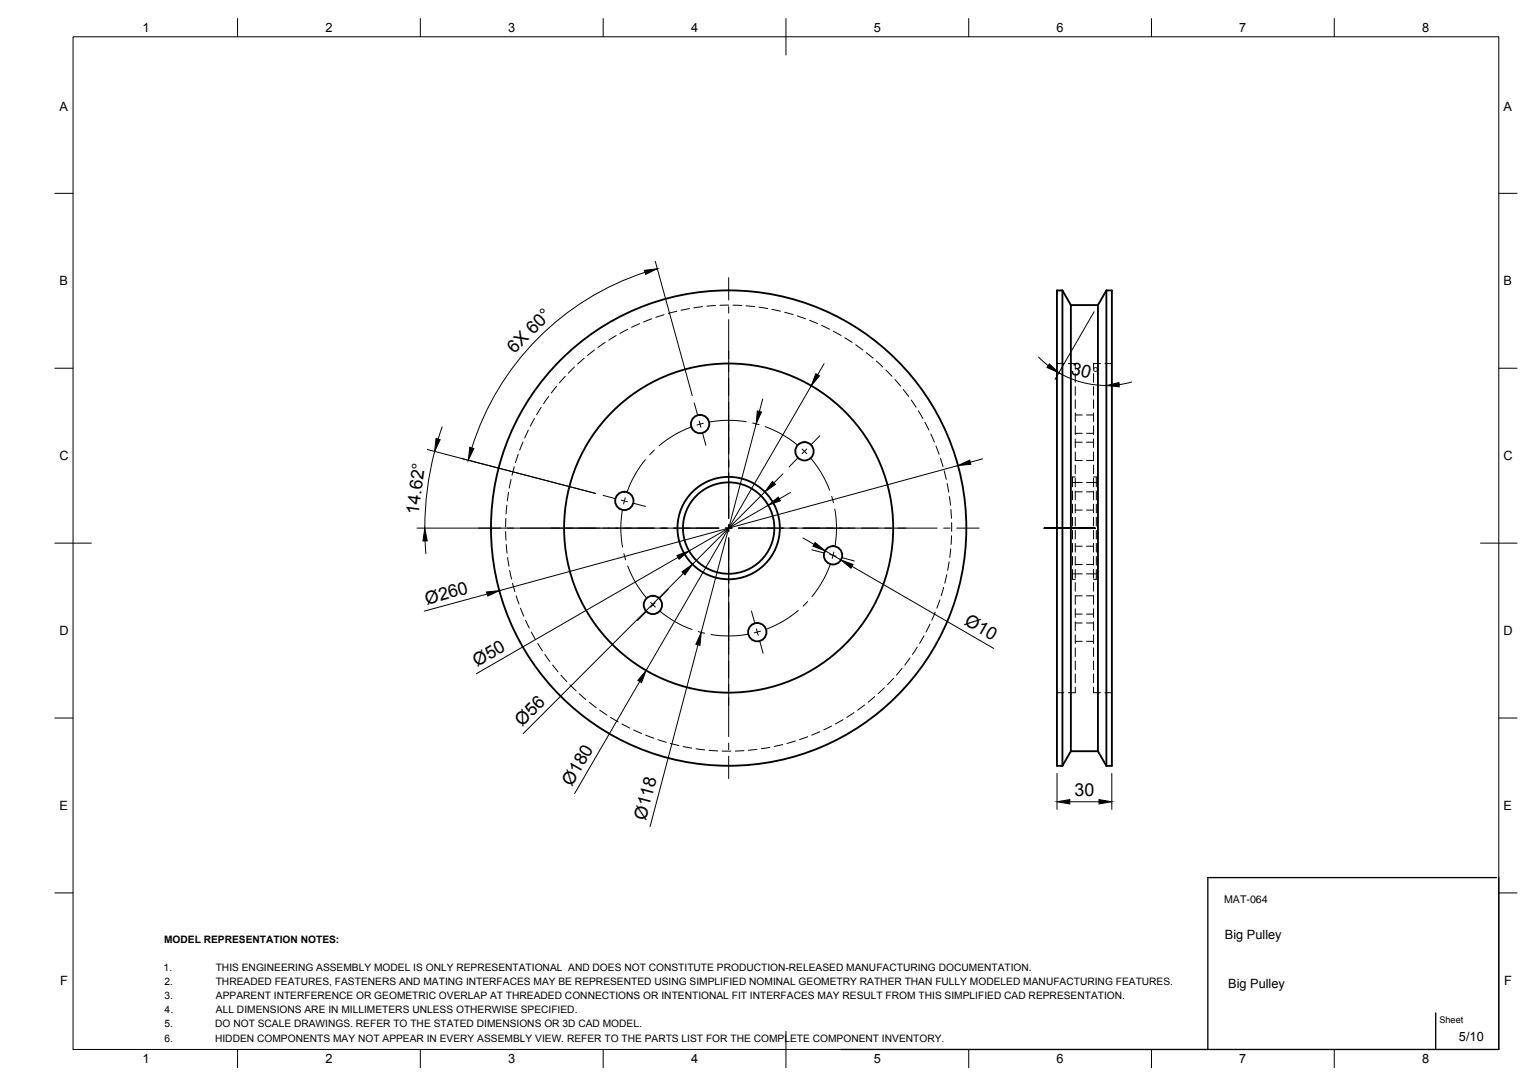
ISO-10303-21;
HEADER;
/* Generated by software containing ST-Developer
 * from STEP Tools, Inc. (www.steptools.com) 
 */

FILE_DESCRIPTION(
/* description */ (''),
/* implementation_level */ '2;1');

FILE_NAME(
/* name */ 
'Big Pulley.step',
/* time_stamp */ '2026-10-24T12:42:14-07:00',
/* author */ (''),
/* organization */ (''),
/* preprocessor_version */ 'ST-DEVELOPER v20.2',
/* originating_system */ 'Autodesk Translation Framework v15.15.0.0',
/* authorisation */ '');

FILE_SCHEMA (('AUTOMOTIVE_DESIGN { 1 0 10303 214 3 1 1 }'));
ENDSEC;

DATA;
#10=MECHANICAL_DESIGN_GEOMETRIC_PRESENTATION_REPRESENTATION('',(#70),#6789);
#16=CONICAL_SURFACE('',#4399,122.,1.04719755119659);
#17=CONICAL_SURFACE('',#4402,130.,1.04719755119659);
#58=SHAPE_REPRESENTATION_RELATIONSHIP('SRR','None',#6825,#64);
#64=ADVANCED_BREP_SHAPE_REPRESENTATION('',(#76),#6787);
#70=STYLED_ITEM('',(#6864),#76);
#76=MANIFOLD_SOLID_BREP('Big Pulley',#3965);
#167=CYLINDRICAL_SURFACE('',#4353,130.);
#168=CYLINDRICAL_SURFACE('',#4356,130.);
#169=CYLINDRICAL_SURFACE('',#4360,5.);
#170=CYLINDRICAL_SURFACE('',#4363,5.);
#171=CYLINDRICAL_SURFACE('',#4366,5.);
#172=CYLINDRICAL_SURFACE('',#4369,5.);
#173=CYLINDRICAL_SURFACE('',#4372,5.);
#174=CYLINDRICAL_SURFACE('',#4375,90.);
#175=CYLINDRICAL_SURFACE('',#4378,90.);
#176=CYLINDRICAL_SURFACE('',#4389,28.);
#177=CYLINDRICAL_SURFACE('',#4391,25.);
#178=CYLINDRICAL_SURFACE('',#4394,28.);
#179=CYLINDRICAL_SURFACE('',#4398,5.);
#180=CYLINDRICAL_SURFACE('',#4404,122.);
#224=FACE_BOUND('',#839,.T.);
#225=FACE_BOUND('',#841,.T.);
#226=FACE_BOUND('',#843,.T.);
#227=FACE_BOUND('',#844,.T.);
#228=FACE_BOUND('',#845,.T.);
#229=FACE_BOUND('',#846,.T.);
#230=FACE_BOUND('',#847,.T.);
#231=FACE_BOUND('',#848,.T.);
#232=FACE_BOUND('',#849,.T.);
#233=FACE_BOUND('',#851,.T.);
#234=FACE_BOUND('',#852,.T.);
#235=FACE_BOUND('',#853,.T.);
#236=FACE_BOUND('',#854,.T.);
#237=FACE_BOUND('',#855,.T.);
#238=FACE_BOUND('',#856,.T.);
#239=FACE_BOUND('',#857,.T.);
#240=FACE_BOUND('',#862,.T.);
#241=FACE_BOUND('',#864,.T.);
#356=CIRCLE('',#4354,130.);
#357=CIRCLE('',#4355,130.);
#358=CIRCLE('',#4357,130.);
#359=CIRCLE('',#4358,130.);
#360=CIRCLE('',#4359,130.);
#361=CIRCLE('',#4361,5.);
#362=CIRCLE('',#4362,5.);
#363=CIRCLE('',#4364,5.);
#364=CIRCLE('',#4365,5.);
#365=CIRCLE('',#4367,5.);
#366=CIRCLE('',#4368,5.);
#367=CIRCLE('',#4370,5.);
#368=CIRCLE('',#4371,5.);
#369=CIRCLE('',#4373,5.);
#370=CIRCLE('',#4374,5.);
#371=CIRCLE('',#4376,90.);
#372=CIRCLE('',#4377,90.);
#373=CIRCLE('',#4379,90.);
#374=CIRCLE('',#4380,90.);
#375=CIRCLE('',#4384,5.);
#376=CIRCLE('',#4385,28.);
#377=CIRCLE('',#4387,5.);
#378=CIRCLE('',#4388,28.);
#379=CIRCLE('',#4390,28.);
#380=CIRCLE('',#4392,25.);
#381=CIRCLE('',#4393,25.);
#382=CIRCLE('',#4395,28.);
#383=CIRCLE('',#4400,122.);
#384=CIRCLE('',#4401,122.);
#385=CIRCLE('',#4403,122.);
#573=FACE_OUTER_BOUND('',#829,.T.);
#574=FACE_OUTER_BOUND('',#830,.T.);
#575=FACE_OUTER_BOUND('',#831,.T.);
#576=FACE_OUTER_BOUND('',#832,.T.);
#577=FACE_OUTER_BOUND('',#833,.T.);
#578=FACE_OUTER_BOUND('',#834,.T.);
#579=FACE_OUTER_BOUND('',#835,.T.);
#580=FACE_OUTER_BOUND('',#836,.T.);
#581=FACE_OUTER_BOUND('',#837,.T.);
#582=FACE_OUTER_BOUND('',#838,.T.);
#583=FACE_OUTER_BOUND('',#840,.T.);
#584=FACE_OUTER_BOUND('',#842,.T.);
#585=FACE_OUTER_BOUND('',#850,.T.);
#586=FACE_OUTER_BOUND('',#858,.T.);
#587=FACE_OUTER_BOUND('',#859,.T.);
#588=FACE_OUTER_BOUND('',#860,.T.);
#589=FACE_OUTER_BOUND('',#861,.T.);
#590=FACE_OUTER_BOUND('',#863,.T.);
#591=FACE_OUTER_BOUND('',#865,.T.);
#592=FACE_OUTER_BOUND('',#866,.T.);
#593=FACE_OUTER_BOUND('',#867,.T.);
#594=FACE_OUTER_BOUND('',#868,.T.);
#829=EDGE_LOOP('',(#3469,#3470,#3471,#3472));
#830=EDGE_LOOP('',(#3473,#3474,#3475,#3476,#3477));
#831=EDGE_LOOP('',(#3478,#3479,#3480,#3481));
#832=EDGE_LOOP('',(#3482,#3483,#3484,#3485));
#833=EDGE_LOOP('',(#3486,#3487,#3488,#3489));
#834=EDGE_LOOP('',(#3490,#3491,#3492,#3493));
#835=EDGE_LOOP('',(#3494,#3495,#3496,#3497));
#836=EDGE_LOOP('',(#3498,#3499,#3500,#3501));
#837=EDGE_LOOP('',(#3502,#3503,#3504,#3505));
#838=EDGE_LOOP('',(#3506));
#839=EDGE_LOOP('',(#3507));
#840=EDGE_LOOP('',(#3508));
#841=EDGE_LOOP('',(#3509));
#842=EDGE_LOOP('',(#3510));
#843=EDGE_LOOP('',(#3511));
#844=EDGE_LOOP('',(#3512));
#845=EDGE_LOOP('',(#3513));
#846=EDGE_LOOP('',(#3514));
#847=EDGE_LOOP('',(#3515));
#848=EDGE_LOOP('',(#3516));
#849=EDGE_LOOP('',(#3517));
#850=EDGE_LOOP('',(#3518));
#851=EDGE_LOOP('',(#3519));
#852=EDGE_LOOP('',(#3520));
#853=EDGE_LOOP('',(#3521));
#854=EDGE_LOOP('',(#3522));
#855=EDGE_LOOP('',(#3523));
#856=EDGE_LOOP('',(#3524));
#857=EDGE_LOOP('',(#3525));
#858=EDGE_LOOP('',(#3526,#3527,#3528,#3529));
#859=EDGE_LOOP('',(#3530,#3531,#3532,#3533));
#860=EDGE_LOOP('',(#3534,#3535,#3536,#3537));
#861=EDGE_LOOP('',(#3538));
#862=EDGE_LOOP('',(#3539));
#863=EDGE_LOOP('',(#3540));
#864=EDGE_LOOP('',(#3541));
#865=EDGE_LOOP('',(#3542,#3543,#3544,#3545));
#866=EDGE_LOOP('',(#3546,#3547,#3548,#3549,#3550));
#867=EDGE_LOOP('',(#3551,#3552,#3553,#3554,#3555));
#868=EDGE_LOOP('',(#3556,#3557,#3558,#3559,#3560));
#1223=LINE('',#6567,#1601);
#1224=LINE('',#6575,#1602);
#1225=LINE('',#6581,#1603);
#1226=LINE('',#6587,#1604);
#1227=LINE('',#6593,#1605);
#1228=LINE('',#6599,#1606);
#1229=LINE('',#6605,#1607);
#1230=LINE('',#6611,#1608);
#1231=LINE('',#6617,#1609);
#1232=LINE('',#6634,#1610);
#1233=LINE('',#6639,#1611);
#1234=LINE('',#6643,#1612);
#1235=LINE('',#6648,#1613);
#1236=LINE('',#6651,#1614);
#1237=LINE('',#6657,#1615);
#1238=LINE('',#6660,#1616);
#1601=VECTOR('',#5412,130.);
#1602=VECTOR('',#5421,130.);
#1603=VECTOR('',#5428,5.);
#1604=VECTOR('',#5435,5.);
#1605=VECTOR('',#5442,5.);
#1606=VECTOR('',#5449,5.);
#1607=VECTOR('',#5456,5.);
#1608=VECTOR('',#5463,90.);
#1609=VECTOR('',#5470,90.);
#1610=VECTOR('',#5493,28.);
#1611=VECTOR('',#5498,25.);
#1612=VECTOR('',#5503,28.);
#1613=VECTOR('',#5512,5.);
#1614=VECTOR('',#5515,122.);
#1615=VECTOR('',#5522,130.);
#1616=VECTOR('',#5527,122.);
#1941=VERTEX_POINT('',#6564);
#1942=VERTEX_POINT('',#6566);
#1943=VERTEX_POINT('',#6570);
#1944=VERTEX_POINT('',#6571);
#1945=VERTEX_POINT('',#6574);
#1946=VERTEX_POINT('',#6578);
#1947=VERTEX_POINT('',#6580);
#1948=VERTEX_POINT('',#6584);
#1949=VERTEX_POINT('',#6586);
#1950=VERTEX_POINT('',#6590);
#1951=VERTEX_POINT('',#6592);
#1952=VERTEX_POINT('',#6596);
#1953=VERTEX_POINT('',#6598);
#1954=VERTEX_POINT('',#6602);
#1955=VERTEX_POINT('',#6604);
#1956=VERTEX_POINT('',#6608);
#1957=VERTEX_POINT('',#6610);
#1958=VERTEX_POINT('',#6614);
#1959=VERTEX_POINT('',#6616);
#1960=VERTEX_POINT('',#6622);
#1961=VERTEX_POINT('',#6624);
#1962=VERTEX_POINT('',#6627);
#1963=VERTEX_POINT('',#6629);
#1964=VERTEX_POINT('',#6632);
#1965=VERTEX_POINT('',#6636);
#1966=VERTEX_POINT('',#6638);
#1967=VERTEX_POINT('',#6642);
#1968=VERTEX_POINT('',#6650);
#1969=VERTEX_POINT('',#6652);
#1970=VERTEX_POINT('',#6656);
#2455=EDGE_CURVE('',#1941,#1941,#356,.T.);
#2456=EDGE_CURVE('',#1941,#1942,#1223,.T.);
#2457=EDGE_CURVE('',#1942,#1942,#357,.T.);
#2458=EDGE_CURVE('',#1943,#1944,#358,.T.);
#2459=EDGE_CURVE('',#1944,#1943,#359,.T.);
#2460=EDGE_CURVE('',#1943,#1945,#1224,.T.);
#2461=EDGE_CURVE('',#1945,#1945,#360,.T.);
#2462=EDGE_CURVE('',#1946,#1946,#361,.T.);
#2463=EDGE_CURVE('',#1946,#1947,#1225,.T.);
#2464=EDGE_CURVE('',#1947,#1947,#362,.T.);
#2465=EDGE_CURVE('',#1948,#1948,#363,.T.);
#2466=EDGE_CURVE('',#1948,#1949,#1226,.T.);
#2467=EDGE_CURVE('',#1949,#1949,#364,.T.);
#2468=EDGE_CURVE('',#1950,#1950,#365,.T.);
#2469=EDGE_CURVE('',#1950,#1951,#1227,.T.);
#2470=EDGE_CURVE('',#1951,#1951,#366,.T.);
#2471=EDGE_CURVE('',#1952,#1952,#367,.T.);
#2472=EDGE_CURVE('',#1952,#1953,#1228,.T.);
#2473=EDGE_CURVE('',#1953,#1953,#368,.T.);
#2474=EDGE_CURVE('',#1954,#1954,#369,.T.);
#2475=EDGE_CURVE('',#1954,#1955,#1229,.T.);
#2476=EDGE_CURVE('',#1955,#1955,#370,.T.);
#2477=EDGE_CURVE('',#1956,#1956,#371,.T.);
#2478=EDGE_CURVE('',#1956,#1957,#1230,.T.);
#2479=EDGE_CURVE('',#1957,#1957,#372,.T.);
#2480=EDGE_CURVE('',#1958,#1958,#373,.T.);
#2481=EDGE_CURVE('',#1958,#1959,#1231,.T.);
#2482=EDGE_CURVE('',#1959,#1959,#374,.T.);
#2483=EDGE_CURVE('',#1960,#1960,#375,.T.);
#2484=EDGE_CURVE('',#1961,#1961,#376,.T.);
#2485=EDGE_CURVE('',#1962,#1962,#377,.T.);
#2486=EDGE_CURVE('',#1963,#1963,#378,.F.);
#2487=EDGE_CURVE('',#1964,#1964,#379,.T.);
#2488=EDGE_CURVE('',#1964,#1963,#1232,.T.);
#2489=EDGE_CURVE('',#1965,#1965,#380,.T.);
#2490=EDGE_CURVE('',#1965,#1966,#1233,.T.);
#2491=EDGE_CURVE('',#1966,#1966,#381,.T.);
#2492=EDGE_CURVE('',#1961,#1967,#1234,.T.);
#2493=EDGE_CURVE('',#1967,#1967,#382,.T.);
#2494=EDGE_CURVE('',#1962,#1960,#1235,.T.);
#2495=EDGE_CURVE('',#1942,#1968,#1236,.T.);
#2496=EDGE_CURVE('',#1969,#1968,#383,.T.);
#2497=EDGE_CURVE('',#1968,#1969,#384,.T.);
#2498=EDGE_CURVE('',#1944,#1970,#1237,.T.);
#2499=EDGE_CURVE('',#1970,#1970,#385,.T.);
#2500=EDGE_CURVE('',#1970,#1969,#1238,.T.);
#3469=ORIENTED_EDGE('',*,*,#2455,.T.);
#3470=ORIENTED_EDGE('',*,*,#2456,.T.);
#3471=ORIENTED_EDGE('',*,*,#2457,.F.);
#3472=ORIENTED_EDGE('',*,*,#2456,.F.);
#3473=ORIENTED_EDGE('',*,*,#2458,.T.);
#3474=ORIENTED_EDGE('',*,*,#2459,.T.);
#3475=ORIENTED_EDGE('',*,*,#2460,.T.);
#3476=ORIENTED_EDGE('',*,*,#2461,.F.);
#3477=ORIENTED_EDGE('',*,*,#2460,.F.);
#3478=ORIENTED_EDGE('',*,*,#2462,.F.);
#3479=ORIENTED_EDGE('',*,*,#2463,.T.);
#3480=ORIENTED_EDGE('',*,*,#2464,.T.);
#3481=ORIENTED_EDGE('',*,*,#2463,.F.);
#3482=ORIENTED_EDGE('',*,*,#2465,.F.);
#3483=ORIENTED_EDGE('',*,*,#2466,.T.);
#3484=ORIENTED_EDGE('',*,*,#2467,.T.);
#3485=ORIENTED_EDGE('',*,*,#2466,.F.);
#3486=ORIENTED_EDGE('',*,*,#2468,.F.);
#3487=ORIENTED_EDGE('',*,*,#2469,.T.);
#3488=ORIENTED_EDGE('',*,*,#2470,.T.);
#3489=ORIENTED_EDGE('',*,*,#2469,.F.);
#3490=ORIENTED_EDGE('',*,*,#2471,.F.);
#3491=ORIENTED_EDGE('',*,*,#2472,.T.);
#3492=ORIENTED_EDGE('',*,*,#2473,.T.);
#3493=ORIENTED_EDGE('',*,*,#2472,.F.);
#3494=ORIENTED_EDGE('',*,*,#2474,.F.);
#3495=ORIENTED_EDGE('',*,*,#2475,.T.);
#3496=ORIENTED_EDGE('',*,*,#2476,.T.);
#3497=ORIENTED_EDGE('',*,*,#2475,.F.);
#3498=ORIENTED_EDGE('',*,*,#2477,.T.);
#3499=ORIENTED_EDGE('',*,*,#2478,.T.);
#3500=ORIENTED_EDGE('',*,*,#2479,.F.);
#3501=ORIENTED_EDGE('',*,*,#2478,.F.);
#3502=ORIENTED_EDGE('',*,*,#2480,.T.);
#3503=ORIENTED_EDGE('',*,*,#2481,.T.);
#3504=ORIENTED_EDGE('',*,*,#2482,.F.);
#3505=ORIENTED_EDGE('',*,*,#2481,.F.);
#3506=ORIENTED_EDGE('',*,*,#2461,.T.);
#3507=ORIENTED_EDGE('',*,*,#2480,.F.);
#3508=ORIENTED_EDGE('',*,*,#2455,.F.);
#3509=ORIENTED_EDGE('',*,*,#2479,.T.);
#3510=ORIENTED_EDGE('',*,*,#2482,.T.);
#3511=ORIENTED_EDGE('',*,*,#2464,.F.);
#3512=ORIENTED_EDGE('',*,*,#2467,.F.);
#3513=ORIENTED_EDGE('',*,*,#2470,.F.);
#3514=ORIENTED_EDGE('',*,*,#2473,.F.);
#3515=ORIENTED_EDGE('',*,*,#2476,.F.);
#3516=ORIENTED_EDGE('',*,*,#2483,.F.);
#3517=ORIENTED_EDGE('',*,*,#2484,.F.);
#3518=ORIENTED_EDGE('',*,*,#2477,.F.);
#3519=ORIENTED_EDGE('',*,*,#2462,.T.);
#3520=ORIENTED_EDGE('',*,*,#2465,.T.);
#3521=ORIENTED_EDGE('',*,*,#2468,.T.);
#3522=ORIENTED_EDGE('',*,*,#2471,.T.);
#3523=ORIENTED_EDGE('',*,*,#2474,.T.);
#3524=ORIENTED_EDGE('',*,*,#2485,.T.);
#3525=ORIENTED_EDGE('',*,*,#2486,.F.);
#3526=ORIENTED_EDGE('',*,*,#2487,.T.);
#3527=ORIENTED_EDGE('',*,*,#2488,.T.);
#3528=ORIENTED_EDGE('',*,*,#2486,.T.);
#3529=ORIENTED_EDGE('',*,*,#2488,.F.);
#3530=ORIENTED_EDGE('',*,*,#2489,.T.);
#3531=ORIENTED_EDGE('',*,*,#2490,.T.);
#3532=ORIENTED_EDGE('',*,*,#2491,.F.);
#3533=ORIENTED_EDGE('',*,*,#2490,.F.);
#3534=ORIENTED_EDGE('',*,*,#2484,.T.);
#3535=ORIENTED_EDGE('',*,*,#2492,.T.);
#3536=ORIENTED_EDGE('',*,*,#2493,.F.);
#3537=ORIENTED_EDGE('',*,*,#2492,.F.);
#3538=ORIENTED_EDGE('',*,*,#2493,.T.);
#3539=ORIENTED_EDGE('',*,*,#2489,.F.);
#3540=ORIENTED_EDGE('',*,*,#2487,.F.);
#3541=ORIENTED_EDGE('',*,*,#2491,.T.);
#3542=ORIENTED_EDGE('',*,*,#2485,.F.);
#3543=ORIENTED_EDGE('',*,*,#2494,.T.);
#3544=ORIENTED_EDGE('',*,*,#2483,.T.);
#3545=ORIENTED_EDGE('',*,*,#2494,.F.);
#3546=ORIENTED_EDGE('',*,*,#2457,.T.);
#3547=ORIENTED_EDGE('',*,*,#2495,.T.);
#3548=ORIENTED_EDGE('',*,*,#2496,.F.);
#3549=ORIENTED_EDGE('',*,*,#2497,.F.);
#3550=ORIENTED_EDGE('',*,*,#2495,.F.);
#3551=ORIENTED_EDGE('',*,*,#2458,.F.);
#3552=ORIENTED_EDGE('',*,*,#2459,.F.);
#3553=ORIENTED_EDGE('',*,*,#2498,.T.);
#3554=ORIENTED_EDGE('',*,*,#2499,.T.);
#3555=ORIENTED_EDGE('',*,*,#2498,.F.);
#3556=ORIENTED_EDGE('',*,*,#2499,.F.);
#3557=ORIENTED_EDGE('',*,*,#2500,.T.);
#3558=ORIENTED_EDGE('',*,*,#2496,.T.);
#3559=ORIENTED_EDGE('',*,*,#2497,.T.);
#3560=ORIENTED_EDGE('',*,*,#2500,.F.);
#3730=PLANE('',#4381);
#3731=PLANE('',#4382);
#3732=PLANE('',#4383);
#3733=PLANE('',#4386);
#3734=PLANE('',#4396);
#3735=PLANE('',#4397);
#3923=ADVANCED_FACE('',(#573),#167,.T.);
#3924=ADVANCED_FACE('',(#574),#168,.T.);
#3925=ADVANCED_FACE('',(#575),#169,.F.);
#3926=ADVANCED_FACE('',(#576),#170,.F.);
#3927=ADVANCED_FACE('',(#577),#171,.F.);
#3928=ADVANCED_FACE('',(#578),#172,.F.);
#3929=ADVANCED_FACE('',(#579),#173,.F.);
#3930=ADVANCED_FACE('',(#580),#174,.F.);
#3931=ADVANCED_FACE('',(#581),#175,.F.);
#3932=ADVANCED_FACE('',(#582,#224),#3730,.T.);
#3933=ADVANCED_FACE('',(#583,#225),#3731,.F.);
#3934=ADVANCED_FACE('',(#584,#226,#227,#228,#229,#230,#231,#232),#3732,
 .T.);
#3935=ADVANCED_FACE('',(#585,#233,#234,#235,#236,#237,#238,#239),#3733,
 .F.);
#3936=ADVANCED_FACE('',(#586),#176,.T.);
#3937=ADVANCED_FACE('',(#587),#177,.F.);
#3938=ADVANCED_FACE('',(#588),#178,.T.);
#3939=ADVANCED_FACE('',(#589,#240),#3734,.T.);
#3940=ADVANCED_FACE('',(#590,#241),#3735,.F.);
#3941=ADVANCED_FACE('',(#591),#179,.F.);
#3942=ADVANCED_FACE('',(#592),#16,.T.);
#3943=ADVANCED_FACE('',(#593),#17,.T.);
#3944=ADVANCED_FACE('',(#594),#180,.T.);
#3965=CLOSED_SHELL('',(#3923,#3924,#3925,#3926,#3927,#3928,#3929,#3930,
#3931,#3932,#3933,#3934,#3935,#3936,#3937,#3938,#3939,#3940,#3941,#3942,
#3943,#3944));
#4352=AXIS2_PLACEMENT_3D('',#6562,#5406,#5407);
#4353=AXIS2_PLACEMENT_3D('',#6563,#5408,#5409);
#4354=AXIS2_PLACEMENT_3D('',#6565,#5410,#5411);
#4355=AXIS2_PLACEMENT_3D('',#6568,#5413,#5414);
#4356=AXIS2_PLACEMENT_3D('',#6569,#5415,#5416);
#4357=AXIS2_PLACEMENT_3D('',#6572,#5417,#5418);
#4358=AXIS2_PLACEMENT_3D('',#6573,#5419,#5420);
#4359=AXIS2_PLACEMENT_3D('',#6576,#5422,#5423);
#4360=AXIS2_PLACEMENT_3D('',#6577,#5424,#5425);
#4361=AXIS2_PLACEMENT_3D('',#6579,#5426,#5427);
#4362=AXIS2_PLACEMENT_3D('',#6582,#5429,#5430);
#4363=AXIS2_PLACEMENT_3D('',#6583,#5431,#5432);
#4364=AXIS2_PLACEMENT_3D('',#6585,#5433,#5434);
#4365=AXIS2_PLACEMENT_3D('',#6588,#5436,#5437);
#4366=AXIS2_PLACEMENT_3D('',#6589,#5438,#5439);
#4367=AXIS2_PLACEMENT_3D('',#6591,#5440,#5441);
#4368=AXIS2_PLACEMENT_3D('',#6594,#5443,#5444);
#4369=AXIS2_PLACEMENT_3D('',#6595,#5445,#5446);
#4370=AXIS2_PLACEMENT_3D('',#6597,#5447,#5448);
#4371=AXIS2_PLACEMENT_3D('',#6600,#5450,#5451);
#4372=AXIS2_PLACEMENT_3D('',#6601,#5452,#5453);
#4373=AXIS2_PLACEMENT_3D('',#6603,#5454,#5455);
#4374=AXIS2_PLACEMENT_3D('',#6606,#5457,#5458);
#4375=AXIS2_PLACEMENT_3D('',#6607,#5459,#5460);
#4376=AXIS2_PLACEMENT_3D('',#6609,#5461,#5462);
#4377=AXIS2_PLACEMENT_3D('',#6612,#5464,#5465);
#4378=AXIS2_PLACEMENT_3D('',#6613,#5466,#5467);
#4379=AXIS2_PLACEMENT_3D('',#6615,#5468,#5469);
#4380=AXIS2_PLACEMENT_3D('',#6618,#5471,#5472);
#4381=AXIS2_PLACEMENT_3D('',#6619,#5473,#5474);
#4382=AXIS2_PLACEMENT_3D('',#6620,#5475,#5476);
#4383=AXIS2_PLACEMENT_3D('',#6621,#5477,#5478);
#4384=AXIS2_PLACEMENT_3D('',#6623,#5479,#5480);
#4385=AXIS2_PLACEMENT_3D('',#6625,#5481,#5482);
#4386=AXIS2_PLACEMENT_3D('',#6626,#5483,#5484);
#4387=AXIS2_PLACEMENT_3D('',#6628,#5485,#5486);
#4388=AXIS2_PLACEMENT_3D('',#6630,#5487,#5488);
#4389=AXIS2_PLACEMENT_3D('',#6631,#5489,#5490);
#4390=AXIS2_PLACEMENT_3D('',#6633,#5491,#5492);
#4391=AXIS2_PLACEMENT_3D('',#6635,#5494,#5495);
#4392=AXIS2_PLACEMENT_3D('',#6637,#5496,#5497);
#4393=AXIS2_PLACEMENT_3D('',#6640,#5499,#5500);
#4394=AXIS2_PLACEMENT_3D('',#6641,#5501,#5502);
#4395=AXIS2_PLACEMENT_3D('',#6644,#5504,#5505);
#4396=AXIS2_PLACEMENT_3D('',#6645,#5506,#5507);
#4397=AXIS2_PLACEMENT_3D('',#6646,#5508,#5509);
#4398=AXIS2_PLACEMENT_3D('',#6647,#5510,#5511);
#4399=AXIS2_PLACEMENT_3D('',#6649,#5513,#5514);
#4400=AXIS2_PLACEMENT_3D('',#6653,#5516,#5517);
#4401=AXIS2_PLACEMENT_3D('',#6654,#5518,#5519);
#4402=AXIS2_PLACEMENT_3D('',#6655,#5520,#5521);
#4403=AXIS2_PLACEMENT_3D('',#6658,#5523,#5524);
#4404=AXIS2_PLACEMENT_3D('',#6659,#5525,#5526);
#5406=DIRECTION('axis',(0.,0.,1.));
#5407=DIRECTION('refdir',(1.,0.,0.));
#5408=DIRECTION('center_axis',(0.,0.,-1.));
#5409=DIRECTION('ref_axis',(-1.,0.,0.));
#5410=DIRECTION('center_axis',(0.,0.,1.));
#5411=DIRECTION('ref_axis',(1.,0.,0.));
#5412=DIRECTION('',(0.,0.,1.));
#5413=DIRECTION('center_axis',(0.,0.,1.));
#5414=DIRECTION('ref_axis',(1.,0.,0.));
#5415=DIRECTION('center_axis',(0.,0.,-1.));
#5416=DIRECTION('ref_axis',(-1.,0.,0.));
#5417=DIRECTION('center_axis',(0.,0.,1.));
#5418=DIRECTION('ref_axis',(1.,0.,0.));
#5419=DIRECTION('center_axis',(0.,0.,1.));
#5420=DIRECTION('ref_axis',(1.,0.,0.));
#5421=DIRECTION('',(0.,0.,1.));
#5422=DIRECTION('center_axis',(0.,0.,1.));
#5423=DIRECTION('ref_axis',(1.,0.,0.));
#5424=DIRECTION('center_axis',(0.,0.,1.));
#5425=DIRECTION('ref_axis',(0.50000000000001,-0.866025403784433,0.));
#5426=DIRECTION('center_axis',(0.,0.,1.));
#5427=DIRECTION('ref_axis',(0.50000000000001,-0.866025403784433,0.));
#5428=DIRECTION('',(0.,0.,1.));
#5429=DIRECTION('center_axis',(0.,0.,1.));
#5430=DIRECTION('ref_axis',(0.50000000000001,-0.866025403784433,0.));
#5431=DIRECTION('center_axis',(0.,0.,1.));
#5432=DIRECTION('ref_axis',(-0.499999999999992,-0.866025403784443,0.));
#5433=DIRECTION('center_axis',(0.,0.,1.));
#5434=DIRECTION('ref_axis',(-0.499999999999992,-0.866025403784443,0.));
#5435=DIRECTION('',(0.,0.,1.));
#5436=DIRECTION('center_axis',(0.,0.,1.));
#5437=DIRECTION('ref_axis',(-0.499999999999992,-0.866025403784443,0.));
#5438=DIRECTION('center_axis',(0.,0.,1.));
#5439=DIRECTION('ref_axis',(-1.,0.,0.));
#5440=DIRECTION('center_axis',(0.,0.,1.));
#5441=DIRECTION('ref_axis',(-1.,0.,0.));
#5442=DIRECTION('',(0.,0.,1.));
#5443=DIRECTION('center_axis',(0.,0.,1.));
#5444=DIRECTION('ref_axis',(-1.,0.,0.));
#5445=DIRECTION('center_axis',(0.,0.,1.));
#5446=DIRECTION('ref_axis',(-0.500000000000004,0.866025403784436,0.));
#5447=DIRECTION('center_axis',(0.,0.,1.));
#5448=DIRECTION('ref_axis',(-0.500000000000004,0.866025403784436,0.));
#5449=DIRECTION('',(0.,0.,1.));
#5450=DIRECTION('center_axis',(0.,0.,1.));
#5451=DIRECTION('ref_axis',(-0.500000000000004,0.866025403784436,0.));
#5452=DIRECTION('center_axis',(0.,0.,1.));
#5453=DIRECTION('ref_axis',(0.499999999999998,0.86602540378444,0.));
#5454=DIRECTION('center_axis',(0.,0.,1.));
#5455=DIRECTION('ref_axis',(0.499999999999998,0.86602540378444,0.));
#5456=DIRECTION('',(0.,0.,1.));
#5457=DIRECTION('center_axis',(0.,0.,1.));
#5458=DIRECTION('ref_axis',(0.499999999999998,0.86602540378444,0.));
#5459=DIRECTION('center_axis',(0.,0.,-1.));
#5460=DIRECTION('ref_axis',(-1.,0.,0.));
#5461=DIRECTION('center_axis',(0.,0.,1.));
#5462=DIRECTION('ref_axis',(1.,0.,0.));
#5463=DIRECTION('',(0.,0.,-1.));
#5464=DIRECTION('center_axis',(0.,0.,1.));
#5465=DIRECTION('ref_axis',(1.,0.,0.));
#5466=DIRECTION('center_axis',(0.,0.,-1.));
#5467=DIRECTION('ref_axis',(-1.,0.,0.));
#5468=DIRECTION('center_axis',(0.,0.,1.));
#5469=DIRECTION('ref_axis',(1.,0.,0.));
#5470=DIRECTION('',(0.,0.,-1.));
#5471=DIRECTION('center_axis',(0.,0.,1.));
#5472=DIRECTION('ref_axis',(1.,0.,0.));
#5473=DIRECTION('center_axis',(0.,0.,1.));
#5474=DIRECTION('ref_axis',(1.,0.,0.));
#5475=DIRECTION('center_axis',(0.,0.,1.));
#5476=DIRECTION('ref_axis',(1.,0.,0.));
#5477=DIRECTION('center_axis',(0.,0.,1.));
#5478=DIRECTION('ref_axis',(1.,0.,0.));
#5479=DIRECTION('center_axis',(0.,0.,1.));
#5480=DIRECTION('ref_axis',(1.,0.,0.));
#5481=DIRECTION('center_axis',(0.,0.,1.));
#5482=DIRECTION('ref_axis',(1.,0.,0.));
#5483=DIRECTION('center_axis',(0.,0.,1.));
#5484=DIRECTION('ref_axis',(1.,0.,0.));
#5485=DIRECTION('center_axis',(0.,0.,1.));
#5486=DIRECTION('ref_axis',(1.,0.,0.));
#5487=DIRECTION('center_axis',(0.,0.,1.));
#5488=DIRECTION('ref_axis',(1.,0.,0.));
#5489=DIRECTION('center_axis',(0.,0.,-1.));
#5490=DIRECTION('ref_axis',(-1.,0.,0.));
#5491=DIRECTION('center_axis',(0.,0.,1.));
#5492=DIRECTION('ref_axis',(1.,0.,0.));
#5493=DIRECTION('',(0.,0.,1.));
#5494=DIRECTION('center_axis',(0.,0.,-1.));
#5495=DIRECTION('ref_axis',(-1.,0.,0.));
#5496=DIRECTION('center_axis',(0.,0.,1.));
#5497=DIRECTION('ref_axis',(1.,0.,0.));
#5498=DIRECTION('',(0.,0.,-1.));
#5499=DIRECTION('center_axis',(0.,0.,1.));
#5500=DIRECTION('ref_axis',(1.,0.,0.));
#5501=DIRECTION('center_axis',(0.,0.,-1.));
#5502=DIRECTION('ref_axis',(-1.,0.,0.));
#5503=DIRECTION('',(0.,0.,1.));
#5504=DIRECTION('center_axis',(0.,0.,1.));
#5505=DIRECTION('ref_axis',(1.,0.,0.));
#5506=DIRECTION('center_axis',(0.,0.,1.));
#5507=DIRECTION('ref_axis',(1.,0.,0.));
#5508=DIRECTION('center_axis',(0.,0.,1.));
#5509=DIRECTION('ref_axis',(1.,0.,0.));
#5510=DIRECTION('center_axis',(0.,0.,1.));
#5511=DIRECTION('ref_axis',(1.,0.,0.));
#5512=DIRECTION('',(0.,0.,1.));
#5513=DIRECTION('center_axis',(0.,0.,-1.));
#5514=DIRECTION('ref_axis',(-1.,0.,0.));
#5515=DIRECTION('',(-0.866025403784436,1.0605752387249E-16,0.500000000000004));
#5516=DIRECTION('center_axis',(0.,0.,1.));
#5517=DIRECTION('ref_axis',(1.,0.,0.));
#5518=DIRECTION('center_axis',(0.,0.,1.));
#5519=DIRECTION('ref_axis',(1.,0.,0.));
#5520=DIRECTION('center_axis',(0.,0.,1.));
#5521=DIRECTION('ref_axis',(1.,0.,0.));
#5522=DIRECTION('',(0.866025403784436,1.0605752387249E-16,-0.500000000000004));
#5523=DIRECTION('center_axis',(0.,0.,1.));
#5524=DIRECTION('ref_axis',(1.,0.,0.));
#5525=DIRECTION('center_axis',(0.,0.,1.));
#5526=DIRECTION('ref_axis',(1.,0.,0.));
#5527=DIRECTION('',(0.,0.,-1.));
#6562=CARTESIAN_POINT('',(0.,0.,0.));
#6563=CARTESIAN_POINT('Origin',(0.,0.,15.));
#6564=CARTESIAN_POINT('',(130.,0.,-15.));
#6565=CARTESIAN_POINT('Origin',(0.,0.,-15.));
#6566=CARTESIAN_POINT('',(130.,0.,-12.));
#6567=CARTESIAN_POINT('',(130.,-1.59204083889156E-14,15.));
#6568=CARTESIAN_POINT('Origin',(0.,0.,-12.));
#6569=CARTESIAN_POINT('Origin',(0.,0.,15.));
#6570=CARTESIAN_POINT('',(130.,0.,12.));
#6571=CARTESIAN_POINT('',(-130.,-1.59204083889156E-14,12.));
#6572=CARTESIAN_POINT('Origin',(0.,0.,12.));
#6573=CARTESIAN_POINT('Origin',(0.,0.,12.));
#6574=CARTESIAN_POINT('',(130.,0.,15.));
#6575=CARTESIAN_POINT('',(130.,-1.59204083889156E-14,15.));
#6576=CARTESIAN_POINT('Origin',(0.,0.,15.));
#6577=CARTESIAN_POINT('Origin',(51.0954988232815,29.5000000000006,-15.));
#6578=CARTESIAN_POINT('',(48.5954988232815,33.8301270189228,-5.));
#6579=CARTESIAN_POINT('Origin',(51.0954988232815,29.5000000000006,-5.));
#6580=CARTESIAN_POINT('',(48.5954988232815,33.8301270189228,5.));
#6581=CARTESIAN_POINT('',(48.5954988232815,33.8301270189228,-15.));
#6582=CARTESIAN_POINT('Origin',(51.0954988232815,29.5000000000006,5.));
#6583=CARTESIAN_POINT('Origin',(51.0954988232822,-29.4999999999995,-15.));
#6584=CARTESIAN_POINT('',(53.5954988232821,-25.1698729810773,-5.));
#6585=CARTESIAN_POINT('Origin',(51.0954988232822,-29.4999999999995,-5.));
#6586=CARTESIAN_POINT('',(53.5954988232821,-25.1698729810773,5.));
#6587=CARTESIAN_POINT('',(53.5954988232821,-25.1698729810773,-15.));
#6588=CARTESIAN_POINT('Origin',(51.0954988232822,-29.4999999999995,5.));
#6589=CARTESIAN_POINT('Origin',(0.,-59.,-15.));
#6590=CARTESIAN_POINT('',(5.,-59.,-5.));
#6591=CARTESIAN_POINT('Origin',(0.,-59.,-5.));
#6592=CARTESIAN_POINT('',(5.,-59.,5.));
#6593=CARTESIAN_POINT('',(5.,-59.,-15.));
#6594=CARTESIAN_POINT('Origin',(0.,-59.,5.));
#6595=CARTESIAN_POINT('Origin',(-51.0954988232818,-29.5000000000002,-15.));
#6596=CARTESIAN_POINT('',(-48.5954988232817,-33.8301270189224,-5.));
#6597=CARTESIAN_POINT('Origin',(-51.0954988232818,-29.5000000000002,-5.));
#6598=CARTESIAN_POINT('',(-48.5954988232817,-33.8301270189224,5.));
#6599=CARTESIAN_POINT('',(-48.5954988232817,-33.8301270189224,-15.));
#6600=CARTESIAN_POINT('Origin',(-51.0954988232818,-29.5000000000002,5.));
#6601=CARTESIAN_POINT('Origin',(-51.095498823282,29.4999999999999,-15.));
#6602=CARTESIAN_POINT('',(-53.5954988232819,25.1698729810777,-5.));
#6603=CARTESIAN_POINT('Origin',(-51.095498823282,29.4999999999999,-5.));
#6604=CARTESIAN_POINT('',(-53.5954988232819,25.1698729810777,5.));
#6605=CARTESIAN_POINT('',(-53.5954988232819,25.1698729810777,-15.));
#6606=CARTESIAN_POINT('Origin',(-51.095498823282,29.4999999999999,5.));
#6607=CARTESIAN_POINT('Origin',(0.,0.,15.));
#6608=CARTESIAN_POINT('',(90.,0.,-5.));
#6609=CARTESIAN_POINT('Origin',(0.,0.,-5.));
#6610=CARTESIAN_POINT('',(90.,0.,-15.));
#6611=CARTESIAN_POINT('',(90.,-1.10218211923262E-14,15.));
#6612=CARTESIAN_POINT('Origin',(0.,0.,-15.));
#6613=CARTESIAN_POINT('Origin',(0.,0.,15.));
#6614=CARTESIAN_POINT('',(90.,0.,15.));
#6615=CARTESIAN_POINT('Origin',(0.,0.,15.));
#6616=CARTESIAN_POINT('',(90.,0.,5.));
#6617=CARTESIAN_POINT('',(90.,-1.10218211923262E-14,15.));
#6618=CARTESIAN_POINT('Origin',(0.,0.,5.));
#6619=CARTESIAN_POINT('Origin',(0.,0.,15.));
#6620=CARTESIAN_POINT('Origin',(0.,0.,-15.));
#6621=CARTESIAN_POINT('Origin',(0.,0.,5.));
#6622=CARTESIAN_POINT('',(-5.,59.,5.));
#6623=CARTESIAN_POINT('Origin',(0.,59.,5.));
#6624=CARTESIAN_POINT('',(28.,0.,5.));
#6625=CARTESIAN_POINT('Origin',(0.,0.,5.));
#6626=CARTESIAN_POINT('Origin',(0.,0.,-5.));
#6627=CARTESIAN_POINT('',(-5.,59.,-5.));
#6628=CARTESIAN_POINT('Origin',(0.,59.,-5.));
#6629=CARTESIAN_POINT('',(28.,0.,-5.));
#6630=CARTESIAN_POINT('Origin',(0.,0.,-5.));
#6631=CARTESIAN_POINT('Origin',(0.,0.,6.5));
#6632=CARTESIAN_POINT('',(28.,0.,-6.5));
#6633=CARTESIAN_POINT('Origin',(0.,0.,-6.5));
#6634=CARTESIAN_POINT('',(28.,-3.42901103761259E-15,6.5));
#6635=CARTESIAN_POINT('Origin',(0.,0.,6.5));
#6636=CARTESIAN_POINT('',(25.,0.,6.5));
#6637=CARTESIAN_POINT('Origin',(0.,0.,6.5));
#6638=CARTESIAN_POINT('',(25.,0.,-6.5));
#6639=CARTESIAN_POINT('',(25.,-3.06161699786838E-15,6.5));
#6640=CARTESIAN_POINT('Origin',(0.,0.,-6.5));
#6641=CARTESIAN_POINT('Origin',(0.,0.,6.5));
#6642=CARTESIAN_POINT('',(28.,0.,6.5));
#6643=CARTESIAN_POINT('',(28.,-3.42901103761259E-15,6.5));
#6644=CARTESIAN_POINT('Origin',(0.,0.,6.5));
#6645=CARTESIAN_POINT('Origin',(0.,0.,6.5));
#6646=CARTESIAN_POINT('Origin',(0.,0.,-6.5));
#6647=CARTESIAN_POINT('Origin',(0.,59.,-15.));
#6648=CARTESIAN_POINT('',(-5.,59.,-15.));
#6649=CARTESIAN_POINT('Origin',(0.,0.,-7.38119784648294));
#6650=CARTESIAN_POINT('',(122.,0.,-7.38119784648294));
#6651=CARTESIAN_POINT('',(122.,-1.49406909495977E-14,-7.38119784648294));
#6652=CARTESIAN_POINT('',(-122.,-1.49406909495977E-14,-7.38119784648294));
#6653=CARTESIAN_POINT('Origin',(0.,0.,-7.38119784648294));
#6654=CARTESIAN_POINT('Origin',(0.,0.,-7.38119784648294));
#6655=CARTESIAN_POINT('Origin',(0.,0.,12.));
#6656=CARTESIAN_POINT('',(-122.,-1.49406909495977E-14,7.38119784648294));
#6657=CARTESIAN_POINT('',(-130.,-1.59204083889156E-14,12.));
#6658=CARTESIAN_POINT('Origin',(0.,0.,7.38119784648294));
#6659=CARTESIAN_POINT('Origin',(0.,0.,15.));
#6660=CARTESIAN_POINT('',(-122.,-1.49406909495977E-14,15.));
#6778=UNCERTAINTY_MEASURE_WITH_UNIT(LENGTH_MEASURE(0.01),#6790,
'DISTANCE_ACCURACY_VALUE',
'Maximum model space distance between geometric entities at asserted c
onnectivities');
#6780=UNCERTAINTY_MEASURE_WITH_UNIT(LENGTH_MEASURE(0.01),#6790,
'DISTANCE_ACCURACY_VALUE',
'Maximum model space distance between geometric entities at asserted c
onnectivities');
#6787=(
GEOMETRIC_REPRESENTATION_CONTEXT(3)
GLOBAL_UNCERTAINTY_ASSIGNED_CONTEXT((#6778))
GLOBAL_UNIT_ASSIGNED_CONTEXT((#6790,#6792,#6793))
REPRESENTATION_CONTEXT('','3D')
);
#6789=(
GEOMETRIC_REPRESENTATION_CONTEXT(3)
GLOBAL_UNCERTAINTY_ASSIGNED_CONTEXT((#6780))
GLOBAL_UNIT_ASSIGNED_CONTEXT((#6790,#6792,#6793))
REPRESENTATION_CONTEXT('','3D')
);
#6790=(
LENGTH_UNIT()
NAMED_UNIT(*)
SI_UNIT(.MILLI.,.METRE.)
);
#6792=(
NAMED_UNIT(*)
PLANE_ANGLE_UNIT()
SI_UNIT($,.RADIAN.)
);
#6793=(
NAMED_UNIT(*)
SI_UNIT($,.STERADIAN.)
SOLID_ANGLE_UNIT()
);
#6800=SHAPE_DEFINITION_REPRESENTATION(#6811,#6825);
#6811=PRODUCT_DEFINITION_SHAPE('',$,#6834);
#6825=SHAPE_REPRESENTATION('',(#4352),#6787);
#6827=PRODUCT_DEFINITION_CONTEXT('part definition',#6853,'design');
#6834=PRODUCT_DEFINITION('Big Pulley','Big Pulley',#6842,#6827);
#6842=PRODUCT_DEFINITION_FORMATION('',$,#6861);
#6853=APPLICATION_CONTEXT(
'Core Data for Automotive Mechanical Design Process');
#6854=PRODUCT_CONTEXT('part definition',#6853,'mechanical');
#6861=PRODUCT('Big Pulley','Big Pulley',$,(#6854));
#6864=PRESENTATION_STYLE_ASSIGNMENT((#6866));
#6866=SURFACE_STYLE_USAGE(.BOTH.,#6868);
#6868=SURFACE_SIDE_STYLE('',(#6870));
#6870=SURFACE_STYLE_FILL_AREA(#6872);
#6872=FILL_AREA_STYLE('Opaque(163,170,173)',(#6874));
#6874=FILL_AREA_STYLE_COLOUR('Opaque(163,170,173)',#6876);
#6876=COLOUR_RGB('Opaque(163,170,173)',0.63921568627451,0.666666666666667,
0.67843137254902);
ENDSEC;
END-ISO-10303-21;
